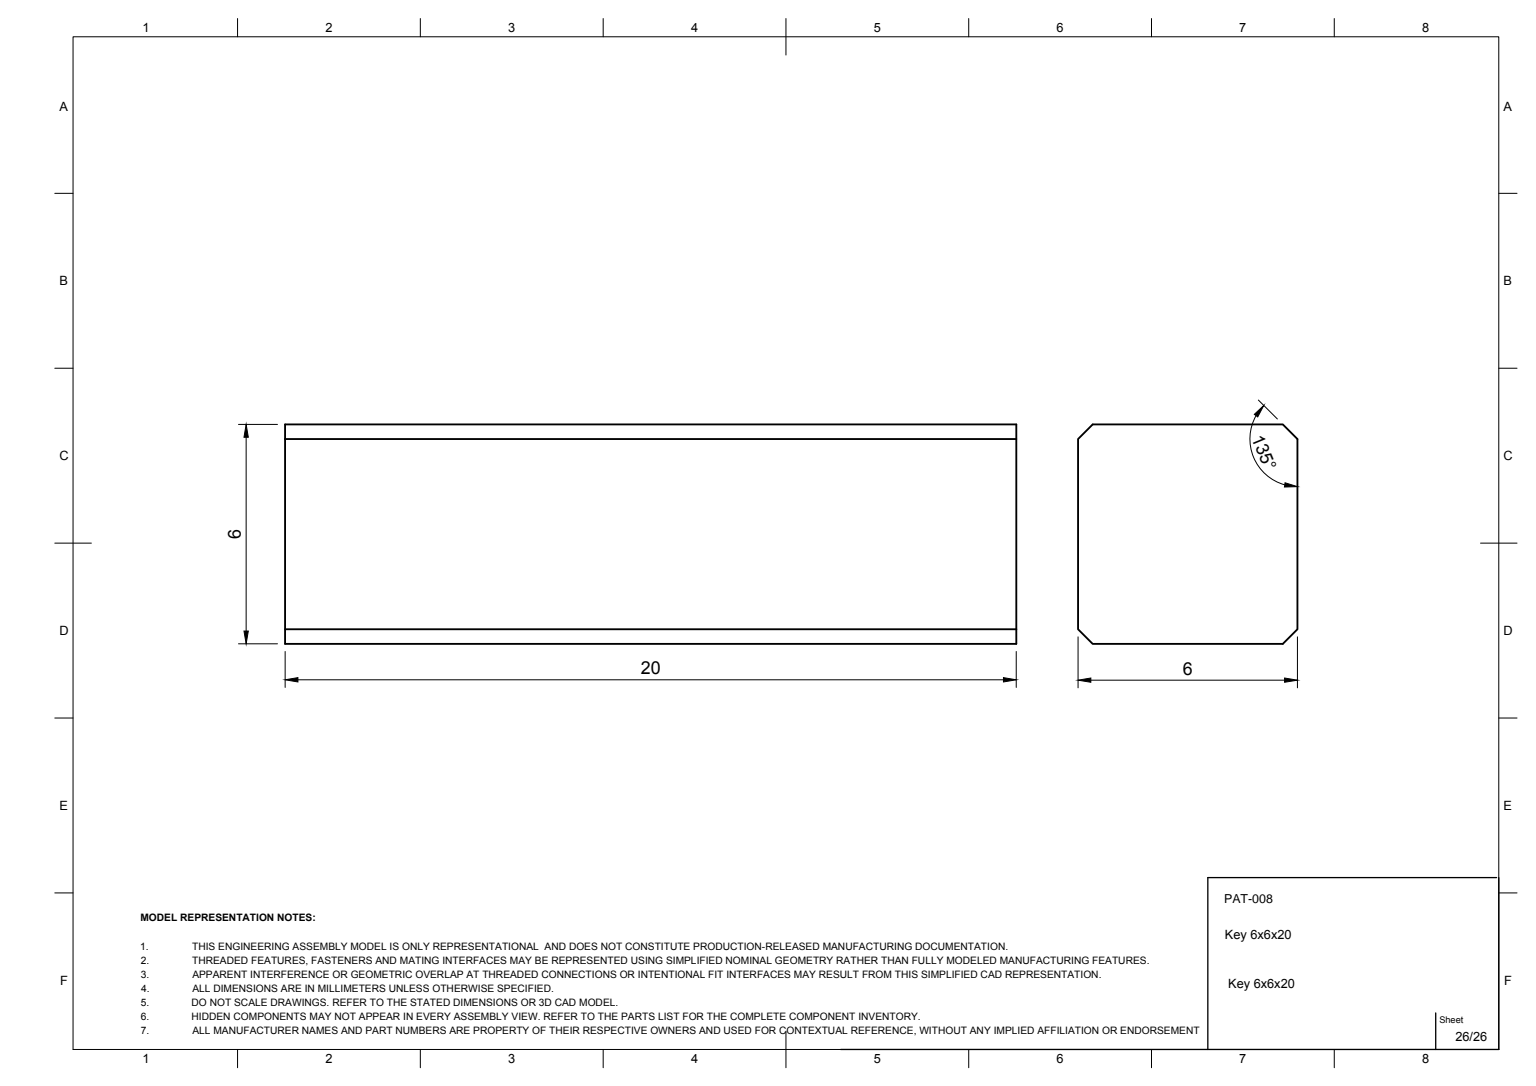
ISO-10303-21;
HEADER;
/* Generated by software containing ST-Developer
 * from STEP Tools, Inc. (www.steptools.com) 
 */

FILE_DESCRIPTION(
/* description */ ('Bearing housing with oil seal and end cap'),
/* implementation_level */ '2;1');

FILE_NAME(
/* name */ 'Key 6x6x20.step',
/* time_stamp */ '2026-10-28T03:23:10-07:00',
/* author */ (''),
/* organization */ (''),
/* preprocessor_version */ 'ST-DEVELOPER v20.2',
/* originating_system */ 'Autodesk Translation Framework v15.17.0.0',
/* authorisation */ '');

FILE_SCHEMA (('AUTOMOTIVE_DESIGN { 1 0 10303 214 3 1 1 }'));
ENDSEC;

DATA;
#10=MECHANICAL_DESIGN_GEOMETRIC_PRESENTATION_REPRESENTATION('',(#286),#7871);
#236=SHAPE_REPRESENTATION_RELATIONSHIP('SRR','None',#7985,#257);
#257=ADVANCED_BREP_SHAPE_REPRESENTATION('',(#313),#7869);
#286=STYLED_ITEM('',(#8153),#313);
#313=MANIFOLD_SOLID_BREP('Body1',#4114);
#533=PLANE('',#4844);
#534=PLANE('',#4845);
#535=PLANE('',#4846);
#536=PLANE('',#4847);
#537=PLANE('',#4848);
#538=PLANE('',#4849);
#539=PLANE('',#4850);
#540=PLANE('',#4851);
#541=PLANE('',#4852);
#542=PLANE('',#4853);
#781=FACE_OUTER_BOUND('',#1124,.T.);
#782=FACE_OUTER_BOUND('',#1125,.T.);
#783=FACE_OUTER_BOUND('',#1126,.T.);
#784=FACE_OUTER_BOUND('',#1127,.T.);
#785=FACE_OUTER_BOUND('',#1128,.T.);
#786=FACE_OUTER_BOUND('',#1129,.T.);
#787=FACE_OUTER_BOUND('',#1130,.T.);
#788=FACE_OUTER_BOUND('',#1131,.T.);
#789=FACE_OUTER_BOUND('',#1132,.T.);
#790=FACE_OUTER_BOUND('',#1133,.T.);
#1124=EDGE_LOOP('',(#3661,#3662,#3663,#3664,#3665,#3666,#3667,#3668));
#1125=EDGE_LOOP('',(#3669,#3670,#3671,#3672));
#1126=EDGE_LOOP('',(#3673,#3674,#3675,#3676));
#1127=EDGE_LOOP('',(#3677,#3678,#3679,#3680));
#1128=EDGE_LOOP('',(#3681,#3682,#3683,#3684));
#1129=EDGE_LOOP('',(#3685,#3686,#3687,#3688,#3689,#3690,#3691,#3692));
#1130=EDGE_LOOP('',(#3693,#3694,#3695,#3696));
#1131=EDGE_LOOP('',(#3697,#3698,#3699,#3700));
#1132=EDGE_LOOP('',(#3701,#3702,#3703,#3704));
#1133=EDGE_LOOP('',(#3705,#3706,#3707,#3708));
#1364=LINE('',#7710,#1626);
#1365=LINE('',#7712,#1627);
#1366=LINE('',#7714,#1628);
#1367=LINE('',#7716,#1629);
#1368=LINE('',#7718,#1630);
#1369=LINE('',#7720,#1631);
#1370=LINE('',#7722,#1632);
#1371=LINE('',#7723,#1633);
#1372=LINE('',#7726,#1634);
#1373=LINE('',#7728,#1635);
#1374=LINE('',#7729,#1636);
#1375=LINE('',#7732,#1637);
#1376=LINE('',#7733,#1638);
#1377=LINE('',#7736,#1639);
#1378=LINE('',#7737,#1640);
#1379=LINE('',#7740,#1641);
#1380=LINE('',#7741,#1642);
#1381=LINE('',#7745,#1643);
#1382=LINE('',#7746,#1644);
#1383=LINE('',#7748,#1645);
#1384=LINE('',#7749,#1646);
#1385=LINE('',#7751,#1647);
#1386=LINE('',#7753,#1648);
#1387=LINE('',#7755,#1649);
#1626=VECTOR('',#6091,1.);
#1627=VECTOR('',#6092,1.);
#1628=VECTOR('',#6093,1.);
#1629=VECTOR('',#6094,1.);
#1630=VECTOR('',#6095,1.);
#1631=VECTOR('',#6096,1.);
#1632=VECTOR('',#6097,1.);
#1633=VECTOR('',#6098,1.);
#1634=VECTOR('',#6101,1.);
#1635=VECTOR('',#6102,1.);
#1636=VECTOR('',#6103,1.);
#1637=VECTOR('',#6106,1.);
#1638=VECTOR('',#6107,1.);
#1639=VECTOR('',#6110,1.);
#1640=VECTOR('',#6111,1.);
#1641=VECTOR('',#6114,1.);
#1642=VECTOR('',#6115,1.);
#1643=VECTOR('',#6118,1.);
#1644=VECTOR('',#6119,1.);
#1645=VECTOR('',#6120,1.);
#1646=VECTOR('',#6121,1.);
#1647=VECTOR('',#6124,1.);
#1648=VECTOR('',#6127,1.);
#1649=VECTOR('',#6130,1.);
#2203=VERTEX_POINT('',#7708);
#2204=VERTEX_POINT('',#7709);
#2205=VERTEX_POINT('',#7711);
#2206=VERTEX_POINT('',#7713);
#2207=VERTEX_POINT('',#7715);
#2208=VERTEX_POINT('',#7717);
#2209=VERTEX_POINT('',#7719);
#2210=VERTEX_POINT('',#7721);
#2211=VERTEX_POINT('',#7725);
#2212=VERTEX_POINT('',#7727);
#2213=VERTEX_POINT('',#7731);
#2214=VERTEX_POINT('',#7735);
#2215=VERTEX_POINT('',#7739);
#2216=VERTEX_POINT('',#7743);
#2217=VERTEX_POINT('',#7744);
#2218=VERTEX_POINT('',#7747);
#2694=EDGE_CURVE('',#2203,#2204,#1364,.T.);
#2695=EDGE_CURVE('',#2205,#2203,#1365,.T.);
#2696=EDGE_CURVE('',#2206,#2205,#1366,.T.);
#2697=EDGE_CURVE('',#2207,#2206,#1367,.T.);
#2698=EDGE_CURVE('',#2208,#2207,#1368,.T.);
#2699=EDGE_CURVE('',#2209,#2208,#1369,.T.);
#2700=EDGE_CURVE('',#2210,#2209,#1370,.T.);
#2701=EDGE_CURVE('',#2204,#2210,#1371,.T.);
#2702=EDGE_CURVE('',#2207,#2211,#1372,.T.);
#2703=EDGE_CURVE('',#2211,#2212,#1373,.T.);
#2704=EDGE_CURVE('',#2212,#2208,#1374,.T.);
#2705=EDGE_CURVE('',#2213,#2206,#1375,.T.);
#2706=EDGE_CURVE('',#2213,#2211,#1376,.T.);
#2707=EDGE_CURVE('',#2205,#2214,#1377,.T.);
#2708=EDGE_CURVE('',#2214,#2213,#1378,.T.);
#2709=EDGE_CURVE('',#2215,#2203,#1379,.T.);
#2710=EDGE_CURVE('',#2215,#2214,#1380,.T.);
#2711=EDGE_CURVE('',#2216,#2217,#1381,.T.);
#2712=EDGE_CURVE('',#2212,#2216,#1382,.T.);
#2713=EDGE_CURVE('',#2218,#2215,#1383,.T.);
#2714=EDGE_CURVE('',#2217,#2218,#1384,.T.);
#2715=EDGE_CURVE('',#2209,#2216,#1385,.T.);
#2716=EDGE_CURVE('',#2204,#2218,#1386,.T.);
#2717=EDGE_CURVE('',#2217,#2210,#1387,.T.);
#3661=ORIENTED_EDGE('',*,*,#2694,.F.);
#3662=ORIENTED_EDGE('',*,*,#2695,.F.);
#3663=ORIENTED_EDGE('',*,*,#2696,.F.);
#3664=ORIENTED_EDGE('',*,*,#2697,.F.);
#3665=ORIENTED_EDGE('',*,*,#2698,.F.);
#3666=ORIENTED_EDGE('',*,*,#2699,.F.);
#3667=ORIENTED_EDGE('',*,*,#2700,.F.);
#3668=ORIENTED_EDGE('',*,*,#2701,.F.);
#3669=ORIENTED_EDGE('',*,*,#2698,.T.);
#3670=ORIENTED_EDGE('',*,*,#2702,.T.);
#3671=ORIENTED_EDGE('',*,*,#2703,.T.);
#3672=ORIENTED_EDGE('',*,*,#2704,.T.);
#3673=ORIENTED_EDGE('',*,*,#2697,.T.);
#3674=ORIENTED_EDGE('',*,*,#2705,.F.);
#3675=ORIENTED_EDGE('',*,*,#2706,.T.);
#3676=ORIENTED_EDGE('',*,*,#2702,.F.);
#3677=ORIENTED_EDGE('',*,*,#2696,.T.);
#3678=ORIENTED_EDGE('',*,*,#2707,.T.);
#3679=ORIENTED_EDGE('',*,*,#2708,.T.);
#3680=ORIENTED_EDGE('',*,*,#2705,.T.);
#3681=ORIENTED_EDGE('',*,*,#2695,.T.);
#3682=ORIENTED_EDGE('',*,*,#2709,.F.);
#3683=ORIENTED_EDGE('',*,*,#2710,.T.);
#3684=ORIENTED_EDGE('',*,*,#2707,.F.);
#3685=ORIENTED_EDGE('',*,*,#2711,.F.);
#3686=ORIENTED_EDGE('',*,*,#2712,.F.);
#3687=ORIENTED_EDGE('',*,*,#2703,.F.);
#3688=ORIENTED_EDGE('',*,*,#2706,.F.);
#3689=ORIENTED_EDGE('',*,*,#2708,.F.);
#3690=ORIENTED_EDGE('',*,*,#2710,.F.);
#3691=ORIENTED_EDGE('',*,*,#2713,.F.);
#3692=ORIENTED_EDGE('',*,*,#2714,.F.);
#3693=ORIENTED_EDGE('',*,*,#2699,.T.);
#3694=ORIENTED_EDGE('',*,*,#2704,.F.);
#3695=ORIENTED_EDGE('',*,*,#2712,.T.);
#3696=ORIENTED_EDGE('',*,*,#2715,.F.);
#3697=ORIENTED_EDGE('',*,*,#2694,.T.);
#3698=ORIENTED_EDGE('',*,*,#2716,.T.);
#3699=ORIENTED_EDGE('',*,*,#2713,.T.);
#3700=ORIENTED_EDGE('',*,*,#2709,.T.);
#3701=ORIENTED_EDGE('',*,*,#2700,.T.);
#3702=ORIENTED_EDGE('',*,*,#2715,.T.);
#3703=ORIENTED_EDGE('',*,*,#2711,.T.);
#3704=ORIENTED_EDGE('',*,*,#2717,.T.);
#3705=ORIENTED_EDGE('',*,*,#2701,.T.);
#3706=ORIENTED_EDGE('',*,*,#2717,.F.);
#3707=ORIENTED_EDGE('',*,*,#2714,.T.);
#3708=ORIENTED_EDGE('',*,*,#2716,.F.);
#4063=ADVANCED_FACE('',(#781),#533,.F.);
#4064=ADVANCED_FACE('',(#782),#534,.T.);
#4065=ADVANCED_FACE('',(#783),#535,.T.);
#4066=ADVANCED_FACE('',(#784),#536,.T.);
#4067=ADVANCED_FACE('',(#785),#537,.T.);
#4068=ADVANCED_FACE('',(#786),#538,.T.);
#4069=ADVANCED_FACE('',(#787),#539,.F.);
#4070=ADVANCED_FACE('',(#788),#540,.T.);
#4071=ADVANCED_FACE('',(#789),#541,.T.);
#4072=ADVANCED_FACE('',(#790),#542,.T.);
#4114=CLOSED_SHELL('',(#4063,#4064,#4065,#4066,#4067,#4068,#4069,#4070,
#4071,#4072));
#4843=AXIS2_PLACEMENT_3D('',#7706,#6087,#6088);
#4844=AXIS2_PLACEMENT_3D('',#7707,#6089,#6090);
#4845=AXIS2_PLACEMENT_3D('',#7724,#6099,#6100);
#4846=AXIS2_PLACEMENT_3D('',#7730,#6104,#6105);
#4847=AXIS2_PLACEMENT_3D('',#7734,#6108,#6109);
#4848=AXIS2_PLACEMENT_3D('',#7738,#6112,#6113);
#4849=AXIS2_PLACEMENT_3D('',#7742,#6116,#6117);
#4850=AXIS2_PLACEMENT_3D('',#7750,#6122,#6123);
#4851=AXIS2_PLACEMENT_3D('',#7752,#6125,#6126);
#4852=AXIS2_PLACEMENT_3D('',#7754,#6128,#6129);
#4853=AXIS2_PLACEMENT_3D('',#7756,#6131,#6132);
#6087=DIRECTION('axis',(0.,0.,1.));
#6088=DIRECTION('refdir',(1.,0.,0.));
#6089=DIRECTION('center_axis',(1.,0.,0.));
#6090=DIRECTION('ref_axis',(0.,0.,-1.));
#6091=DIRECTION('',(0.,-0.707106781186547,-0.707106781186548));
#6092=DIRECTION('',(0.,-1.,0.));
#6093=DIRECTION('',(0.,-0.707106781186547,0.707106781186548));
#6094=DIRECTION('',(0.,0.,1.));
#6095=DIRECTION('',(0.,0.707106781186547,0.707106781186548));
#6096=DIRECTION('',(0.,1.,0.));
#6097=DIRECTION('',(0.,0.707106781186547,-0.707106781186548));
#6098=DIRECTION('',(0.,0.,-1.));
#6099=DIRECTION('center_axis',(0.,0.707106781186548,-0.707106781186547));
#6100=DIRECTION('ref_axis',(-1.,0.,0.));
#6101=DIRECTION('',(1.,0.,0.));
#6102=DIRECTION('',(0.,-0.707106781186547,-0.707106781186548));
#6103=DIRECTION('',(-1.,0.,0.));
#6104=DIRECTION('center_axis',(0.,1.,0.));
#6105=DIRECTION('ref_axis',(-1.,0.,0.));
#6106=DIRECTION('',(-1.,0.,0.));
#6107=DIRECTION('',(0.,0.,-1.));
#6108=DIRECTION('center_axis',(0.,0.707106781186548,0.707106781186547));
#6109=DIRECTION('ref_axis',(1.,0.,0.));
#6110=DIRECTION('',(1.,0.,0.));
#6111=DIRECTION('',(0.,0.707106781186547,-0.707106781186548));
#6112=DIRECTION('center_axis',(0.,0.,1.));
#6113=DIRECTION('ref_axis',(1.,0.,0.));
#6114=DIRECTION('',(-1.,0.,0.));
#6115=DIRECTION('',(0.,1.,0.));
#6116=DIRECTION('center_axis',(1.,0.,0.));
#6117=DIRECTION('ref_axis',(0.,0.,-1.));
#6118=DIRECTION('',(0.,-0.707106781186547,0.707106781186548));
#6119=DIRECTION('',(0.,-1.,0.));
#6120=DIRECTION('',(0.,0.707106781186547,0.707106781186548));
#6121=DIRECTION('',(0.,0.,1.));
#6122=DIRECTION('center_axis',(0.,0.,1.));
#6123=DIRECTION('ref_axis',(1.,0.,0.));
#6124=DIRECTION('',(1.,0.,0.));
#6125=DIRECTION('center_axis',(0.,-0.707106781186548,0.707106781186547));
#6126=DIRECTION('ref_axis',(1.,0.,0.));
#6127=DIRECTION('',(1.,0.,0.));
#6128=DIRECTION('center_axis',(0.,-0.707106781186548,-0.707106781186547));
#6129=DIRECTION('ref_axis',(-1.,0.,0.));
#6130=DIRECTION('',(-1.,0.,0.));
#6131=DIRECTION('center_axis',(0.,-1.,0.));
#6132=DIRECTION('ref_axis',(1.,0.,0.));
#7706=CARTESIAN_POINT('',(0.,0.,0.));
#7707=CARTESIAN_POINT('Origin',(-1.,0.,0.35));
#7708=CARTESIAN_POINT('',(-1.,-0.26,0.6));
#7709=CARTESIAN_POINT('',(-1.,-0.3,0.56));
#7710=CARTESIAN_POINT('',(-1.,-0.2675,0.5925));
#7711=CARTESIAN_POINT('',(-1.,0.26,0.6));
#7712=CARTESIAN_POINT('',(-1.,0.,0.6));
#7713=CARTESIAN_POINT('',(-1.,0.3,0.56));
#7714=CARTESIAN_POINT('',(-1.,0.2675,0.5925));
#7715=CARTESIAN_POINT('',(-1.,0.3,0.04));
#7716=CARTESIAN_POINT('',(-1.,0.3,0.175));
#7717=CARTESIAN_POINT('',(-1.,0.26,0.));
#7718=CARTESIAN_POINT('',(-1.,0.2925,0.0325));
#7719=CARTESIAN_POINT('',(-1.,-0.26,0.));
#7720=CARTESIAN_POINT('',(-1.,0.,0.));
#7721=CARTESIAN_POINT('',(-1.,-0.3,0.04));
#7722=CARTESIAN_POINT('',(-1.,-0.2925,0.0325));
#7723=CARTESIAN_POINT('',(-1.,-0.3,0.175));
#7724=CARTESIAN_POINT('Origin',(0.75,0.28,0.02));
#7725=CARTESIAN_POINT('',(1.,0.3,0.04));
#7726=CARTESIAN_POINT('',(0.75,0.3,0.04));
#7727=CARTESIAN_POINT('',(1.,0.26,0.));
#7728=CARTESIAN_POINT('',(1.,0.2925,0.0325));
#7729=CARTESIAN_POINT('',(0.75,0.26,0.));
#7730=CARTESIAN_POINT('Origin',(1.5,0.3,0.));
#7731=CARTESIAN_POINT('',(1.,0.3,0.56));
#7732=CARTESIAN_POINT('',(0.75,0.3,0.56));
#7733=CARTESIAN_POINT('',(1.,0.3,0.175));
#7734=CARTESIAN_POINT('Origin',(0.75,0.28,0.58));
#7735=CARTESIAN_POINT('',(1.,0.26,0.6));
#7736=CARTESIAN_POINT('',(0.75,0.26,0.6));
#7737=CARTESIAN_POINT('',(1.,0.2675,0.5925));
#7738=CARTESIAN_POINT('Origin',(0.,0.,0.6));
#7739=CARTESIAN_POINT('',(1.,-0.26,0.6));
#7740=CARTESIAN_POINT('',(-0.75,-0.26,0.6));
#7741=CARTESIAN_POINT('',(1.,0.,0.6));
#7742=CARTESIAN_POINT('Origin',(1.,0.,0.35));
#7743=CARTESIAN_POINT('',(1.,-0.26,0.));
#7744=CARTESIAN_POINT('',(1.,-0.3,0.04));
#7745=CARTESIAN_POINT('',(1.,-0.2925,0.0325));
#7746=CARTESIAN_POINT('',(1.,0.,0.));
#7747=CARTESIAN_POINT('',(1.,-0.3,0.56));
#7748=CARTESIAN_POINT('',(1.,-0.2675,0.5925));
#7749=CARTESIAN_POINT('',(1.,-0.3,0.175));
#7750=CARTESIAN_POINT('Origin',(0.,0.,0.));
#7751=CARTESIAN_POINT('',(-0.75,-0.26,0.));
#7752=CARTESIAN_POINT('Origin',(-0.75,-0.28,0.58));
#7753=CARTESIAN_POINT('',(-0.75,-0.3,0.56));
#7754=CARTESIAN_POINT('Origin',(-0.75,-0.28,0.02));
#7755=CARTESIAN_POINT('',(-0.75,-0.3,0.04));
#7756=CARTESIAN_POINT('Origin',(-1.5,-0.3,0.));
#7843=UNCERTAINTY_MEASURE_WITH_UNIT(LENGTH_MEASURE(0.001),#7872,
'DISTANCE_ACCURACY_VALUE',
'Maximum model space distance between geometric entities at asserted c
onnectivities');
#7845=UNCERTAINTY_MEASURE_WITH_UNIT(LENGTH_MEASURE(0.001),#7872,
'DISTANCE_ACCURACY_VALUE',
'Maximum model space distance between geometric entities at asserted c
onnectivities');
#7869=(
GEOMETRIC_REPRESENTATION_CONTEXT(3)
GLOBAL_UNCERTAINTY_ASSIGNED_CONTEXT((#7843))
GLOBAL_UNIT_ASSIGNED_CONTEXT((#7872,#7874,#7875))
REPRESENTATION_CONTEXT('','3D')
);
#7871=(
GEOMETRIC_REPRESENTATION_CONTEXT(3)
GLOBAL_UNCERTAINTY_ASSIGNED_CONTEXT((#7845))
GLOBAL_UNIT_ASSIGNED_CONTEXT((#7872,#7874,#7875))
REPRESENTATION_CONTEXT('','3D')
);
#7872=(
LENGTH_UNIT()
NAMED_UNIT(*)
SI_UNIT(.CENTI.,.METRE.)
);
#7874=(
NAMED_UNIT(*)
PLANE_ANGLE_UNIT()
SI_UNIT($,.RADIAN.)
);
#7875=(
NAMED_UNIT(*)
SI_UNIT($,.STERADIAN.)
SOLID_ANGLE_UNIT()
);
#7899=SHAPE_DEFINITION_REPRESENTATION(#7951,#7985);
#7951=PRODUCT_DEFINITION_SHAPE('',$,#8011);
#7985=SHAPE_REPRESENTATION('',(#4843),#7869);
#7987=PRODUCT_DEFINITION_CONTEXT('part definition',#8064,'design');
#8011=PRODUCT_DEFINITION('Key 6x6x20','Key 6x6x20',#8036,#7987);
#8036=PRODUCT_DEFINITION_FORMATION('',$,#8089);
#8064=APPLICATION_CONTEXT(
'Core Data for Automotive Mechanical Design Process');
#8065=PRODUCT_CONTEXT('part definition',#8064,'mechanical');
#8089=PRODUCT('Key 6x6x20','Key 6x6x20','Key 6x6x20',(#8065));
#8147=COLOUR_RGB('Grey',0.48,0.52,0.57);
#8148=FILL_AREA_STYLE_COLOUR('',#8147);
#8149=FILL_AREA_STYLE('',(#8148));
#8150=SURFACE_STYLE_FILL_AREA(#8149);
#8151=SURFACE_SIDE_STYLE('',(#8150));
#8152=SURFACE_STYLE_USAGE(.BOTH.,#8151);
#8153=PRESENTATION_STYLE_ASSIGNMENT((#8152));
ENDSEC;
END-ISO-10303-21;
